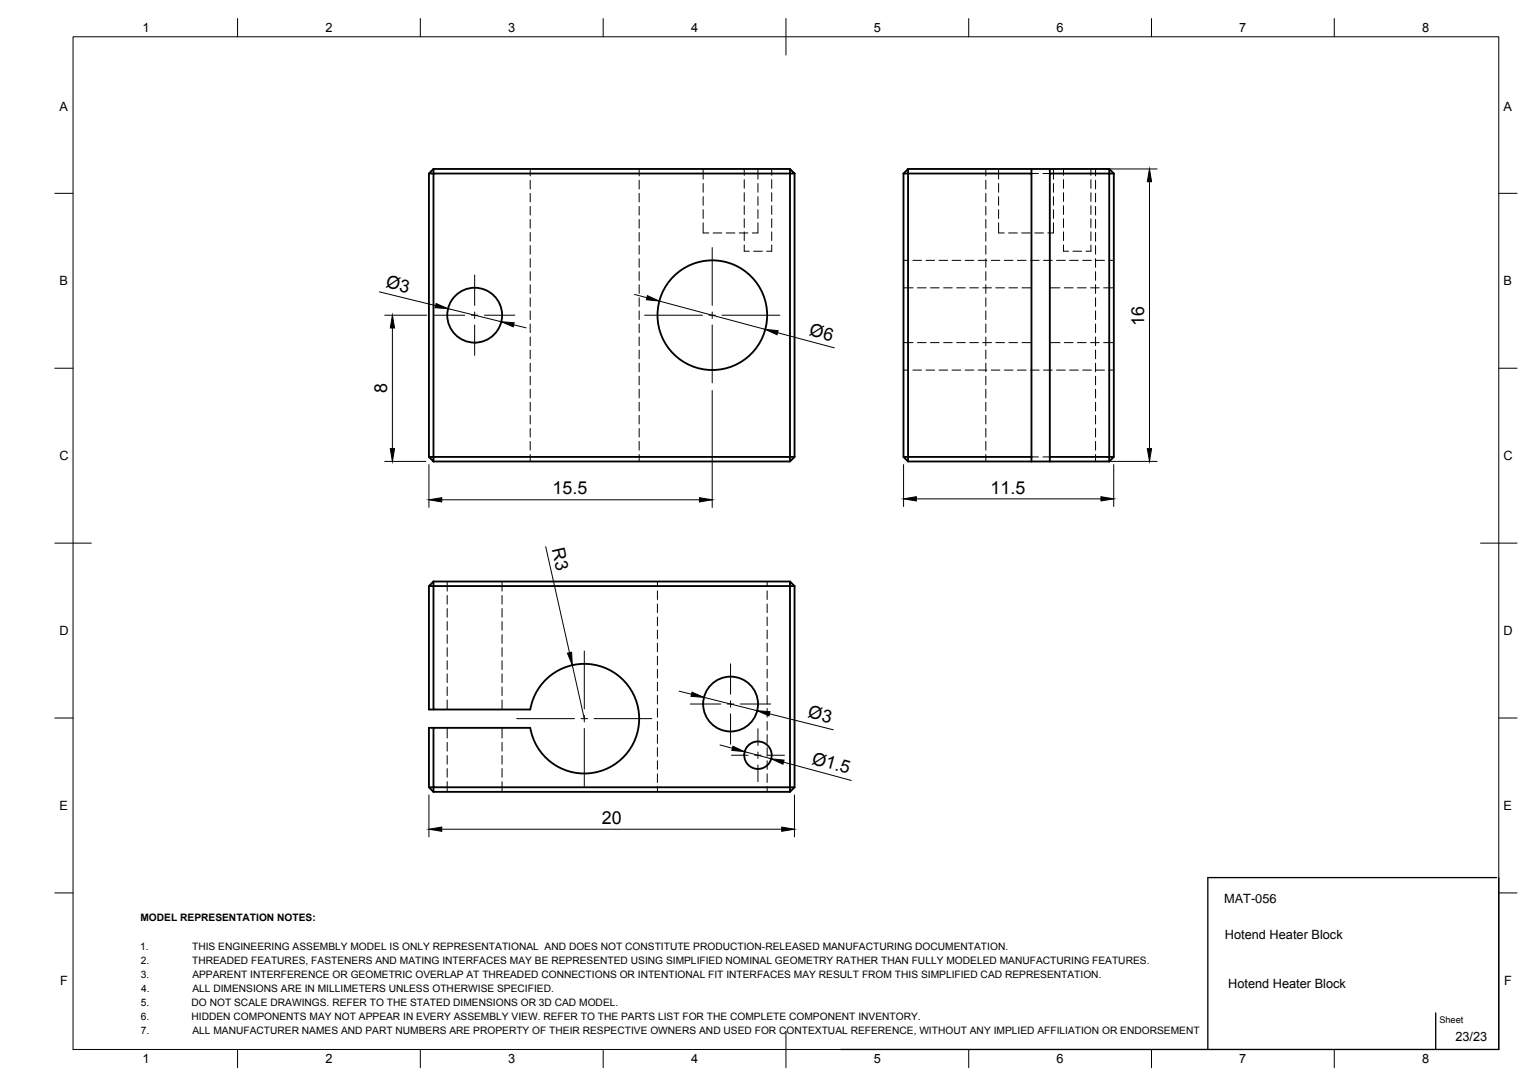
ISO-10303-21;
HEADER;
/* Generated by software containing ST-Developer
 * from STEP Tools, Inc. (www.steptools.com) 
 */

FILE_DESCRIPTION(
/* description */ (''),
/* implementation_level */ '2;1');

FILE_NAME(
/* name */ 'Hotend Heater Block.step',
/* time_stamp */ '2026-10-28T16:47:13+01:00',
/* author */ (''),
/* organization */ (''),
/* preprocessor_version */ 'ST-DEVELOPER v20.2',
/* originating_system */ 'Autodesk Translation Framework v15.17.0.0',
/* authorisation */ '');

FILE_SCHEMA (('AUTOMOTIVE_DESIGN { 1 0 10303 214 3 1 1 }'));
ENDSEC;

DATA;
#10=MECHANICAL_DESIGN_GEOMETRIC_PRESENTATION_REPRESENTATION('',(#4613),#459242);
#4425=SHAPE_REPRESENTATION_RELATIONSHIP('SRR','None',#459352,#4446);
#4446=ADVANCED_BREP_SHAPE_REPRESENTATION('',(#4493),#459241);
#4493=MANIFOLD_SOLID_BREP('E3D V6 heatblock',#94671);
#4613=STYLED_ITEM('',(#459505),#4493);
#5270=FACE_BOUND('',#18094,.T.);
#5271=FACE_BOUND('',#18095,.T.);
#5272=FACE_BOUND('',#18099,.T.);
#5273=FACE_BOUND('',#18100,.T.);
#5274=FACE_BOUND('',#18102,.T.);
#5275=FACE_BOUND('',#18103,.T.);
#5276=FACE_BOUND('',#18105,.T.);
#5277=FACE_BOUND('',#18107,.T.);
#6148=PLANE('',#105513);
#6149=PLANE('',#105514);
#6150=PLANE('',#105515);
#6151=PLANE('',#105516);
#6152=PLANE('',#105517);
#6153=PLANE('',#105518);
#6154=PLANE('',#105519);
#6155=PLANE('',#105520);
#6156=PLANE('',#105521);
#6157=PLANE('',#105522);
#6158=PLANE('',#105523);
#6159=PLANE('',#105524);
#6160=PLANE('',#105525);
#6161=PLANE('',#105526);
#6162=PLANE('',#105527);
#6163=PLANE('',#105528);
#6164=PLANE('',#105529);
#6165=PLANE('',#105530);
#6166=PLANE('',#105531);
#6167=PLANE('',#105532);
#6168=PLANE('',#105533);
#6169=PLANE('',#105534);
#6170=PLANE('',#105535);
#6171=PLANE('',#105536);
#6172=PLANE('',#105537);
#6173=PLANE('',#105538);
#6174=PLANE('',#105539);
#6175=PLANE('',#105540);
#6176=PLANE('',#105541);
#6177=PLANE('',#105542);
#6178=PLANE('',#105543);
#6179=PLANE('',#105544);
#6180=PLANE('',#105545);
#12120=FACE_OUTER_BOUND('',#18085,.T.);
#12121=FACE_OUTER_BOUND('',#18086,.T.);
#12122=FACE_OUTER_BOUND('',#18087,.T.);
#12123=FACE_OUTER_BOUND('',#18088,.T.);
#12124=FACE_OUTER_BOUND('',#18089,.T.);
#12125=FACE_OUTER_BOUND('',#18090,.T.);
#12126=FACE_OUTER_BOUND('',#18091,.T.);
#12127=FACE_OUTER_BOUND('',#18092,.T.);
#12128=FACE_OUTER_BOUND('',#18093,.T.);
#12129=FACE_OUTER_BOUND('',#18096,.T.);
#12130=FACE_OUTER_BOUND('',#18097,.T.);
#12131=FACE_OUTER_BOUND('',#18098,.T.);
#12132=FACE_OUTER_BOUND('',#18101,.T.);
#12133=FACE_OUTER_BOUND('',#18104,.T.);
#12134=FACE_OUTER_BOUND('',#18106,.T.);
#12135=FACE_OUTER_BOUND('',#18108,.T.);
#12136=FACE_OUTER_BOUND('',#18109,.T.);
#12137=FACE_OUTER_BOUND('',#18110,.T.);
#12138=FACE_OUTER_BOUND('',#18111,.T.);
#12139=FACE_OUTER_BOUND('',#18112,.T.);
#12140=FACE_OUTER_BOUND('',#18113,.T.);
#12141=FACE_OUTER_BOUND('',#18114,.T.);
#12142=FACE_OUTER_BOUND('',#18115,.T.);
#12143=FACE_OUTER_BOUND('',#18116,.T.);
#12144=FACE_OUTER_BOUND('',#18117,.T.);
#12145=FACE_OUTER_BOUND('',#18118,.T.);
#12146=FACE_OUTER_BOUND('',#18119,.T.);
#12147=FACE_OUTER_BOUND('',#18120,.T.);
#12148=FACE_OUTER_BOUND('',#18121,.T.);
#12149=FACE_OUTER_BOUND('',#18122,.T.);
#12150=FACE_OUTER_BOUND('',#18123,.T.);
#12151=FACE_OUTER_BOUND('',#18124,.T.);
#12152=FACE_OUTER_BOUND('',#18125,.T.);
#12153=FACE_OUTER_BOUND('',#18126,.T.);
#12154=FACE_OUTER_BOUND('',#18127,.T.);
#12155=FACE_OUTER_BOUND('',#18128,.T.);
#12156=FACE_OUTER_BOUND('',#18129,.T.);
#12157=FACE_OUTER_BOUND('',#18130,.T.);
#12158=FACE_OUTER_BOUND('',#18131,.T.);
#18085=EDGE_LOOP('',(#86890,#86891,#86892,#86893));
#18086=EDGE_LOOP('',(#86894,#86895,#86896,#86897));
#18087=EDGE_LOOP('',(#86898,#86899,#86900,#86901));
#18088=EDGE_LOOP('',(#86902,#86903,#86904,#86905));
#18089=EDGE_LOOP('',(#86906,#86907,#86908,#86909));
#18090=EDGE_LOOP('',(#86910,#86911,#86912,#86913));
#18091=EDGE_LOOP('',(#86914,#86915,#86916,#86917));
#18092=EDGE_LOOP('',(#86918,#86919,#86920,#86921));
#18093=EDGE_LOOP('',(#86922,#86923,#86924,#86925,#86926,#86927,#86928,#86929));
#18094=EDGE_LOOP('',(#86930));
#18095=EDGE_LOOP('',(#86931));
#18096=EDGE_LOOP('',(#86932,#86933,#86934,#86935));
#18097=EDGE_LOOP('',(#86936,#86937,#86938,#86939,#86940,#86941,#86942,#86943));
#18098=EDGE_LOOP('',(#86944,#86945,#86946,#86947));
#18099=EDGE_LOOP('',(#86948));
#18100=EDGE_LOOP('',(#86949));
#18101=EDGE_LOOP('',(#86950,#86951,#86952,#86953));
#18102=EDGE_LOOP('',(#86954));
#18103=EDGE_LOOP('',(#86955));
#18104=EDGE_LOOP('',(#86956,#86957,#86958,#86959,#86960,#86961));
#18105=EDGE_LOOP('',(#86962));
#18106=EDGE_LOOP('',(#86963,#86964,#86965,#86966,#86967,#86968));
#18107=EDGE_LOOP('',(#86969));
#18108=EDGE_LOOP('',(#86970));
#18109=EDGE_LOOP('',(#86971));
#18110=EDGE_LOOP('',(#86972,#86973,#86974,#86975));
#18111=EDGE_LOOP('',(#86976,#86977,#86978,#86979));
#18112=EDGE_LOOP('',(#86980,#86981,#86982));
#18113=EDGE_LOOP('',(#86983,#86984,#86985));
#18114=EDGE_LOOP('',(#86986,#86987,#86988,#86989));
#18115=EDGE_LOOP('',(#86990,#86991,#86992,#86993));
#18116=EDGE_LOOP('',(#86994,#86995,#86996,#86997));
#18117=EDGE_LOOP('',(#86998,#86999,#87000,#87001));
#18118=EDGE_LOOP('',(#87002,#87003,#87004,#87005));
#18119=EDGE_LOOP('',(#87006,#87007,#87008,#87009));
#18120=EDGE_LOOP('',(#87010,#87011,#87012,#87013));
#18121=EDGE_LOOP('',(#87014,#87015,#87016));
#18122=EDGE_LOOP('',(#87017,#87018,#87019));
#18123=EDGE_LOOP('',(#87020,#87021,#87022));
#18124=EDGE_LOOP('',(#87023,#87024,#87025));
#18125=EDGE_LOOP('',(#87026,#87027,#87028,#87029));
#18126=EDGE_LOOP('',(#87030,#87031,#87032,#87033));
#18127=EDGE_LOOP('',(#87034,#87035,#87036,#87037));
#18128=EDGE_LOOP('',(#87038,#87039,#87040,#87041));
#18129=EDGE_LOOP('',(#87042,#87043,#87044));
#18130=EDGE_LOOP('',(#87045,#87046,#87047));
#18131=EDGE_LOOP('',(#87048,#87049,#87050,#87051));
#23486=CIRCLE('',#105496,3.);
#23487=CIRCLE('',#105497,3.);
#23488=CIRCLE('',#105499,1.5);
#23489=CIRCLE('',#105500,1.5);
#23490=CIRCLE('',#105502,1.5);
#23491=CIRCLE('',#105503,1.5);
#23492=CIRCLE('',#105505,0.750000000000001);
#23493=CIRCLE('',#105506,0.750000000000001);
#23494=CIRCLE('',#105508,1.5);
#23495=CIRCLE('',#105509,1.5);
#23496=CIRCLE('',#105511,3.);
#23497=CIRCLE('',#105512,3.);
#30780=LINE('',#459000,#34582);
#30781=LINE('',#459006,#34583);
#30782=LINE('',#459012,#34584);
#30783=LINE('',#459018,#34585);
#30784=LINE('',#459024,#34586);
#30785=LINE('',#459031,#34587);
#30786=LINE('',#459034,#34588);
#30787=LINE('',#459038,#34589);
#30788=LINE('',#459040,#34590);
#30789=LINE('',#459042,#34591);
#30790=LINE('',#459043,#34592);
#30791=LINE('',#459047,#34593);
#30792=LINE('',#459049,#34594);
#30793=LINE('',#459051,#34595);
#30794=LINE('',#459052,#34596);
#30795=LINE('',#459055,#34597);
#30796=LINE('',#459057,#34598);
#30797=LINE('',#459059,#34599);
#30798=LINE('',#459061,#34600);
#30799=LINE('',#459063,#34601);
#30800=LINE('',#459065,#34602);
#30801=LINE('',#459066,#34603);
#30802=LINE('',#459070,#34604);
#30803=LINE('',#459072,#34605);
#30804=LINE('',#459074,#34606);
#30805=LINE('',#459075,#34607);
#30806=LINE('',#459079,#34608);
#30807=LINE('',#459081,#34609);
#30808=LINE('',#459082,#34610);
#30809=LINE('',#459084,#34611);
#30810=LINE('',#459086,#34612);
#30811=LINE('',#459088,#34613);
#30812=LINE('',#459089,#34614);
#30813=LINE('',#459093,#34615);
#30814=LINE('',#459095,#34616);
#30815=LINE('',#459097,#34617);
#30816=LINE('',#459098,#34618);
#30817=LINE('',#459102,#34619);
#30818=LINE('',#459104,#34620);
#30819=LINE('',#459106,#34621);
#30820=LINE('',#459107,#34622);
#30821=LINE('',#459109,#34623);
#30822=LINE('',#459110,#34624);
#30823=LINE('',#459112,#34625);
#30824=LINE('',#459113,#34626);
#30825=LINE('',#459117,#34627);
#30826=LINE('',#459119,#34628);
#30827=LINE('',#459121,#34629);
#30828=LINE('',#459122,#34630);
#30829=LINE('',#459124,#34631);
#30830=LINE('',#459125,#34632);
#30831=LINE('',#459127,#34633);
#30832=LINE('',#459129,#34634);
#30833=LINE('',#459131,#34635);
#30834=LINE('',#459133,#34636);
#30835=LINE('',#459134,#34637);
#30836=LINE('',#459136,#34638);
#30837=LINE('',#459138,#34639);
#30838=LINE('',#459140,#34640);
#30839=LINE('',#459142,#34641);
#30840=LINE('',#459144,#34642);
#30841=LINE('',#459146,#34643);
#30842=LINE('',#459148,#34644);
#30843=LINE('',#459150,#34645);
#30844=LINE('',#459152,#34646);
#30845=LINE('',#459154,#34647);
#30846=LINE('',#459156,#34648);
#30847=LINE('',#459158,#34649);
#30848=LINE('',#459160,#34650);
#34582=VECTOR('',#130494,3.);
#34583=VECTOR('',#130501,1.5);
#34584=VECTOR('',#130508,1.5);
#34585=VECTOR('',#130515,0.750000000000001);
#34586=VECTOR('',#130522,1.5);
#34587=VECTOR('',#130529,1000.);
#34588=VECTOR('',#130532,1000.);
#34589=VECTOR('',#130535,1000.);
#34590=VECTOR('',#130536,1000.);
#34591=VECTOR('',#130537,1000.);
#34592=VECTOR('',#130538,1000.);
#34593=VECTOR('',#130541,1000.);
#34594=VECTOR('',#130542,1000.);
#34595=VECTOR('',#130543,1000.);
#34596=VECTOR('',#130544,1000.);
#34597=VECTOR('',#130547,1000.);
#34598=VECTOR('',#130548,1000.);
#34599=VECTOR('',#130549,1000.);
#34600=VECTOR('',#130550,1000.);
#34601=VECTOR('',#130551,1000.);
#34602=VECTOR('',#130552,1000.);
#34603=VECTOR('',#130553,1000.);
#34604=VECTOR('',#130556,1000.);
#34605=VECTOR('',#130557,1000.);
#34606=VECTOR('',#130558,1000.);
#34607=VECTOR('',#130559,1000.);
#34608=VECTOR('',#130562,1000.);
#34609=VECTOR('',#130563,1000.);
#34610=VECTOR('',#130564,1000.);
#34611=VECTOR('',#130565,1000.);
#34612=VECTOR('',#130566,1000.);
#34613=VECTOR('',#130567,1000.);
#34614=VECTOR('',#130568,1000.);
#34615=VECTOR('',#130571,1000.);
#34616=VECTOR('',#130572,1000.);
#34617=VECTOR('',#130573,1000.);
#34618=VECTOR('',#130574,1000.);
#34619=VECTOR('',#130577,1000.);
#34620=VECTOR('',#130578,1000.);
#34621=VECTOR('',#130579,1000.);
#34622=VECTOR('',#130580,1000.);
#34623=VECTOR('',#130583,1000.);
#34624=VECTOR('',#130584,1000.);
#34625=VECTOR('',#130587,1000.);
#34626=VECTOR('',#130588,1000.);
#34627=VECTOR('',#130595,1000.);
#34628=VECTOR('',#130598,1000.);
#34629=VECTOR('',#130601,1000.);
#34630=VECTOR('',#130602,1000.);
#34631=VECTOR('',#130605,1000.);
#34632=VECTOR('',#130606,1000.);
#34633=VECTOR('',#130609,1000.);
#34634=VECTOR('',#130612,1000.);
#34635=VECTOR('',#130615,1000.);
#34636=VECTOR('',#130618,1000.);
#34637=VECTOR('',#130619,1000.);
#34638=VECTOR('',#130622,1000.);
#34639=VECTOR('',#130625,1000.);
#34640=VECTOR('',#130628,1000.);
#34641=VECTOR('',#130631,1000.);
#34642=VECTOR('',#130634,1000.);
#34643=VECTOR('',#130637,1000.);
#34644=VECTOR('',#130640,1000.);
#34645=VECTOR('',#130643,1000.);
#34646=VECTOR('',#130646,1000.);
#34647=VECTOR('',#130649,1000.);
#34648=VECTOR('',#130652,1000.);
#34649=VECTOR('',#130655,1000.);
#34650=VECTOR('',#130658,1000.);
#43470=VERTEX_POINT('',#458997);
#43471=VERTEX_POINT('',#458999);
#43472=VERTEX_POINT('',#459003);
#43473=VERTEX_POINT('',#459005);
#43474=VERTEX_POINT('',#459009);
#43475=VERTEX_POINT('',#459011);
#43476=VERTEX_POINT('',#459015);
#43477=VERTEX_POINT('',#459017);
#43478=VERTEX_POINT('',#459021);
#43479=VERTEX_POINT('',#459023);
#43480=VERTEX_POINT('',#459027);
#43481=VERTEX_POINT('',#459028);
#43482=VERTEX_POINT('',#459030);
#43483=VERTEX_POINT('',#459032);
#43484=VERTEX_POINT('',#459036);
#43485=VERTEX_POINT('',#459037);
#43486=VERTEX_POINT('',#459039);
#43487=VERTEX_POINT('',#459041);
#43488=VERTEX_POINT('',#459045);
#43489=VERTEX_POINT('',#459046);
#43490=VERTEX_POINT('',#459048);
#43491=VERTEX_POINT('',#459050);
#43492=VERTEX_POINT('',#459054);
#43493=VERTEX_POINT('',#459056);
#43494=VERTEX_POINT('',#459058);
#43495=VERTEX_POINT('',#459060);
#43496=VERTEX_POINT('',#459062);
#43497=VERTEX_POINT('',#459064);
#43498=VERTEX_POINT('',#459068);
#43499=VERTEX_POINT('',#459069);
#43500=VERTEX_POINT('',#459071);
#43501=VERTEX_POINT('',#459073);
#43502=VERTEX_POINT('',#459077);
#43503=VERTEX_POINT('',#459078);
#43504=VERTEX_POINT('',#459080);
#43505=VERTEX_POINT('',#459083);
#43506=VERTEX_POINT('',#459085);
#43507=VERTEX_POINT('',#459087);
#43508=VERTEX_POINT('',#459091);
#43509=VERTEX_POINT('',#459092);
#43510=VERTEX_POINT('',#459094);
#43511=VERTEX_POINT('',#459096);
#43512=VERTEX_POINT('',#459100);
#43513=VERTEX_POINT('',#459101);
#43514=VERTEX_POINT('',#459103);
#43515=VERTEX_POINT('',#459105);
#57947=EDGE_CURVE('',#43470,#43470,#23486,.T.);
#57948=EDGE_CURVE('',#43470,#43471,#30780,.T.);
#57949=EDGE_CURVE('',#43471,#43471,#23487,.T.);
#57950=EDGE_CURVE('',#43472,#43472,#23488,.T.);
#57951=EDGE_CURVE('',#43472,#43473,#30781,.T.);
#57952=EDGE_CURVE('',#43473,#43473,#23489,.T.);
#57953=EDGE_CURVE('',#43474,#43474,#23490,.T.);
#57954=EDGE_CURVE('',#43474,#43475,#30782,.T.);
#57955=EDGE_CURVE('',#43475,#43475,#23491,.T.);
#57956=EDGE_CURVE('',#43476,#43476,#23492,.T.);
#57957=EDGE_CURVE('',#43476,#43477,#30783,.T.);
#57958=EDGE_CURVE('',#43477,#43477,#23493,.T.);
#57959=EDGE_CURVE('',#43478,#43478,#23494,.T.);
#57960=EDGE_CURVE('',#43478,#43479,#30784,.T.);
#57961=EDGE_CURVE('',#43479,#43479,#23495,.T.);
#57962=EDGE_CURVE('',#43480,#43481,#23496,.T.);
#57963=EDGE_CURVE('',#43480,#43482,#30785,.T.);
#57964=EDGE_CURVE('',#43482,#43483,#23497,.T.);
#57965=EDGE_CURVE('',#43481,#43483,#30786,.T.);
#57966=EDGE_CURVE('',#43484,#43485,#30787,.T.);
#57967=EDGE_CURVE('',#43485,#43486,#30788,.T.);
#57968=EDGE_CURVE('',#43487,#43486,#30789,.T.);
#57969=EDGE_CURVE('',#43487,#43484,#30790,.T.);
#57970=EDGE_CURVE('',#43488,#43489,#30791,.T.);
#57971=EDGE_CURVE('',#43489,#43490,#30792,.T.);
#57972=EDGE_CURVE('',#43490,#43491,#30793,.T.);
#57973=EDGE_CURVE('',#43491,#43488,#30794,.T.);
#57974=EDGE_CURVE('',#43492,#43482,#30795,.T.);
#57975=EDGE_CURVE('',#43492,#43493,#30796,.T.);
#57976=EDGE_CURVE('',#43493,#43494,#30797,.T.);
#57977=EDGE_CURVE('',#43494,#43495,#30798,.T.);
#57978=EDGE_CURVE('',#43495,#43496,#30799,.T.);
#57979=EDGE_CURVE('',#43496,#43497,#30800,.T.);
#57980=EDGE_CURVE('',#43483,#43497,#30801,.T.);
#57981=EDGE_CURVE('',#43498,#43499,#30802,.T.);
#57982=EDGE_CURVE('',#43499,#43500,#30803,.T.);
#57983=EDGE_CURVE('',#43500,#43501,#30804,.T.);
#57984=EDGE_CURVE('',#43501,#43498,#30805,.T.);
#57985=EDGE_CURVE('',#43502,#43503,#30806,.T.);
#57986=EDGE_CURVE('',#43503,#43504,#30807,.T.);
#57987=EDGE_CURVE('',#43504,#43480,#30808,.T.);
#57988=EDGE_CURVE('',#43481,#43505,#30809,.T.);
#57989=EDGE_CURVE('',#43505,#43506,#30810,.T.);
#57990=EDGE_CURVE('',#43506,#43507,#30811,.T.);
#57991=EDGE_CURVE('',#43507,#43502,#30812,.T.);
#57992=EDGE_CURVE('',#43508,#43509,#30813,.T.);
#57993=EDGE_CURVE('',#43509,#43510,#30814,.T.);
#57994=EDGE_CURVE('',#43510,#43511,#30815,.T.);
#57995=EDGE_CURVE('',#43511,#43508,#30816,.T.);
#57996=EDGE_CURVE('',#43512,#43513,#30817,.T.);
#57997=EDGE_CURVE('',#43513,#43514,#30818,.T.);
#57998=EDGE_CURVE('',#43514,#43515,#30819,.T.);
#57999=EDGE_CURVE('',#43515,#43512,#30820,.T.);
#58000=EDGE_CURVE('',#43486,#43492,#30821,.T.);
#58001=EDGE_CURVE('',#43504,#43487,#30822,.T.);
#58002=EDGE_CURVE('',#43497,#43489,#30823,.T.);
#58003=EDGE_CURVE('',#43488,#43505,#30824,.T.);
#58004=EDGE_CURVE('',#43506,#43491,#30825,.T.);
#58005=EDGE_CURVE('',#43484,#43503,#30826,.T.);
#58006=EDGE_CURVE('',#43506,#43511,#30827,.T.);
#58007=EDGE_CURVE('',#43511,#43491,#30828,.T.);
#58008=EDGE_CURVE('',#43484,#43512,#30829,.T.);
#58009=EDGE_CURVE('',#43512,#43503,#30830,.T.);
#58010=EDGE_CURVE('',#43490,#43496,#30831,.T.);
#58011=EDGE_CURVE('',#43508,#43490,#30832,.T.);
#58012=EDGE_CURVE('',#43507,#43510,#30833,.T.);
#58013=EDGE_CURVE('',#43502,#43501,#30834,.T.);
#58014=EDGE_CURVE('',#43498,#43507,#30835,.T.);
#58015=EDGE_CURVE('',#43513,#43502,#30836,.T.);
#58016=EDGE_CURVE('',#43485,#43515,#30837,.T.);
#58017=EDGE_CURVE('',#43493,#43485,#30838,.T.);
#58018=EDGE_CURVE('',#43508,#43496,#30839,.T.);
#58019=EDGE_CURVE('',#43498,#43510,#30840,.T.);
#58020=EDGE_CURVE('',#43513,#43501,#30841,.T.);
#58021=EDGE_CURVE('',#43493,#43515,#30842,.T.);
#58022=EDGE_CURVE('',#43509,#43495,#30843,.T.);
#58023=EDGE_CURVE('',#43499,#43509,#30844,.T.);
#58024=EDGE_CURVE('',#43514,#43500,#30845,.T.);
#58025=EDGE_CURVE('',#43494,#43514,#30846,.T.);
#58026=EDGE_CURVE('',#43499,#43495,#30847,.T.);
#58027=EDGE_CURVE('',#43494,#43500,#30848,.T.);
#86890=ORIENTED_EDGE('',*,*,#57947,.F.);
#86891=ORIENTED_EDGE('',*,*,#57948,.T.);
#86892=ORIENTED_EDGE('',*,*,#57949,.T.);
#86893=ORIENTED_EDGE('',*,*,#57948,.F.);
#86894=ORIENTED_EDGE('',*,*,#57950,.F.);
#86895=ORIENTED_EDGE('',*,*,#57951,.T.);
#86896=ORIENTED_EDGE('',*,*,#57952,.F.);
#86897=ORIENTED_EDGE('',*,*,#57951,.F.);
#86898=ORIENTED_EDGE('',*,*,#57953,.F.);
#86899=ORIENTED_EDGE('',*,*,#57954,.T.);
#86900=ORIENTED_EDGE('',*,*,#57955,.T.);
#86901=ORIENTED_EDGE('',*,*,#57954,.F.);
#86902=ORIENTED_EDGE('',*,*,#57956,.F.);
#86903=ORIENTED_EDGE('',*,*,#57957,.T.);
#86904=ORIENTED_EDGE('',*,*,#57958,.T.);
#86905=ORIENTED_EDGE('',*,*,#57957,.F.);
#86906=ORIENTED_EDGE('',*,*,#57959,.F.);
#86907=ORIENTED_EDGE('',*,*,#57960,.T.);
#86908=ORIENTED_EDGE('',*,*,#57961,.T.);
#86909=ORIENTED_EDGE('',*,*,#57960,.F.);
#86910=ORIENTED_EDGE('',*,*,#57962,.F.);
#86911=ORIENTED_EDGE('',*,*,#57963,.T.);
#86912=ORIENTED_EDGE('',*,*,#57964,.T.);
#86913=ORIENTED_EDGE('',*,*,#57965,.F.);
#86914=ORIENTED_EDGE('',*,*,#57966,.T.);
#86915=ORIENTED_EDGE('',*,*,#57967,.T.);
#86916=ORIENTED_EDGE('',*,*,#57968,.F.);
#86917=ORIENTED_EDGE('',*,*,#57969,.T.);
#86918=ORIENTED_EDGE('',*,*,#57970,.T.);
#86919=ORIENTED_EDGE('',*,*,#57971,.T.);
#86920=ORIENTED_EDGE('',*,*,#57972,.T.);
#86921=ORIENTED_EDGE('',*,*,#57973,.T.);
#86922=ORIENTED_EDGE('',*,*,#57974,.F.);
#86923=ORIENTED_EDGE('',*,*,#57975,.T.);
#86924=ORIENTED_EDGE('',*,*,#57976,.T.);
#86925=ORIENTED_EDGE('',*,*,#57977,.T.);
#86926=ORIENTED_EDGE('',*,*,#57978,.T.);
#86927=ORIENTED_EDGE('',*,*,#57979,.T.);
#86928=ORIENTED_EDGE('',*,*,#57980,.F.);
#86929=ORIENTED_EDGE('',*,*,#57964,.F.);
#86930=ORIENTED_EDGE('',*,*,#57958,.F.);
#86931=ORIENTED_EDGE('',*,*,#57961,.F.);
#86932=ORIENTED_EDGE('',*,*,#57981,.T.);
#86933=ORIENTED_EDGE('',*,*,#57982,.T.);
#86934=ORIENTED_EDGE('',*,*,#57983,.T.);
#86935=ORIENTED_EDGE('',*,*,#57984,.T.);
#86936=ORIENTED_EDGE('',*,*,#57985,.T.);
#86937=ORIENTED_EDGE('',*,*,#57986,.T.);
#86938=ORIENTED_EDGE('',*,*,#57987,.T.);
#86939=ORIENTED_EDGE('',*,*,#57962,.T.);
#86940=ORIENTED_EDGE('',*,*,#57988,.T.);
#86941=ORIENTED_EDGE('',*,*,#57989,.T.);
#86942=ORIENTED_EDGE('',*,*,#57990,.T.);
#86943=ORIENTED_EDGE('',*,*,#57991,.T.);
#86944=ORIENTED_EDGE('',*,*,#57992,.T.);
#86945=ORIENTED_EDGE('',*,*,#57993,.T.);
#86946=ORIENTED_EDGE('',*,*,#57994,.T.);
#86947=ORIENTED_EDGE('',*,*,#57995,.T.);
#86948=ORIENTED_EDGE('',*,*,#57949,.F.);
#86949=ORIENTED_EDGE('',*,*,#57955,.F.);
#86950=ORIENTED_EDGE('',*,*,#57996,.T.);
#86951=ORIENTED_EDGE('',*,*,#57997,.T.);
#86952=ORIENTED_EDGE('',*,*,#57998,.T.);
#86953=ORIENTED_EDGE('',*,*,#57999,.T.);
#86954=ORIENTED_EDGE('',*,*,#57947,.T.);
#86955=ORIENTED_EDGE('',*,*,#57950,.T.);
#86956=ORIENTED_EDGE('',*,*,#57968,.T.);
#86957=ORIENTED_EDGE('',*,*,#58000,.T.);
#86958=ORIENTED_EDGE('',*,*,#57974,.T.);
#86959=ORIENTED_EDGE('',*,*,#57963,.F.);
#86960=ORIENTED_EDGE('',*,*,#57987,.F.);
#86961=ORIENTED_EDGE('',*,*,#58001,.T.);
#86962=ORIENTED_EDGE('',*,*,#57952,.T.);
#86963=ORIENTED_EDGE('',*,*,#57980,.T.);
#86964=ORIENTED_EDGE('',*,*,#58002,.T.);
#86965=ORIENTED_EDGE('',*,*,#57970,.F.);
#86966=ORIENTED_EDGE('',*,*,#58003,.T.);
#86967=ORIENTED_EDGE('',*,*,#57988,.F.);
#86968=ORIENTED_EDGE('',*,*,#57965,.T.);
#86969=ORIENTED_EDGE('',*,*,#57953,.T.);
#86970=ORIENTED_EDGE('',*,*,#57959,.T.);
#86971=ORIENTED_EDGE('',*,*,#57956,.T.);
#86972=ORIENTED_EDGE('',*,*,#58003,.F.);
#86973=ORIENTED_EDGE('',*,*,#57973,.F.);
#86974=ORIENTED_EDGE('',*,*,#58004,.F.);
#86975=ORIENTED_EDGE('',*,*,#57989,.F.);
#86976=ORIENTED_EDGE('',*,*,#58001,.F.);
#86977=ORIENTED_EDGE('',*,*,#57986,.F.);
#86978=ORIENTED_EDGE('',*,*,#58005,.F.);
#86979=ORIENTED_EDGE('',*,*,#57969,.F.);
#86980=ORIENTED_EDGE('',*,*,#58006,.F.);
#86981=ORIENTED_EDGE('',*,*,#58004,.T.);
#86982=ORIENTED_EDGE('',*,*,#58007,.F.);
#86983=ORIENTED_EDGE('',*,*,#58008,.F.);
#86984=ORIENTED_EDGE('',*,*,#58005,.T.);
#86985=ORIENTED_EDGE('',*,*,#58009,.F.);
#86986=ORIENTED_EDGE('',*,*,#58002,.F.);
#86987=ORIENTED_EDGE('',*,*,#57979,.F.);
#86988=ORIENTED_EDGE('',*,*,#58010,.F.);
#86989=ORIENTED_EDGE('',*,*,#57971,.F.);
#86990=ORIENTED_EDGE('',*,*,#58007,.T.);
#86991=ORIENTED_EDGE('',*,*,#57972,.F.);
#86992=ORIENTED_EDGE('',*,*,#58011,.F.);
#86993=ORIENTED_EDGE('',*,*,#57995,.F.);
#86994=ORIENTED_EDGE('',*,*,#58006,.T.);
#86995=ORIENTED_EDGE('',*,*,#57994,.F.);
#86996=ORIENTED_EDGE('',*,*,#58012,.F.);
#86997=ORIENTED_EDGE('',*,*,#57990,.F.);
#86998=ORIENTED_EDGE('',*,*,#58013,.F.);
#86999=ORIENTED_EDGE('',*,*,#57991,.F.);
#87000=ORIENTED_EDGE('',*,*,#58014,.F.);
#87001=ORIENTED_EDGE('',*,*,#57984,.F.);
#87002=ORIENTED_EDGE('',*,*,#58009,.T.);
#87003=ORIENTED_EDGE('',*,*,#57985,.F.);
#87004=ORIENTED_EDGE('',*,*,#58015,.F.);
#87005=ORIENTED_EDGE('',*,*,#57996,.F.);
#87006=ORIENTED_EDGE('',*,*,#58008,.T.);
#87007=ORIENTED_EDGE('',*,*,#57999,.F.);
#87008=ORIENTED_EDGE('',*,*,#58016,.F.);
#87009=ORIENTED_EDGE('',*,*,#57966,.F.);
#87010=ORIENTED_EDGE('',*,*,#58000,.F.);
#87011=ORIENTED_EDGE('',*,*,#57967,.F.);
#87012=ORIENTED_EDGE('',*,*,#58017,.F.);
#87013=ORIENTED_EDGE('',*,*,#57975,.F.);
#87014=ORIENTED_EDGE('',*,*,#58011,.T.);
#87015=ORIENTED_EDGE('',*,*,#58010,.T.);
#87016=ORIENTED_EDGE('',*,*,#58018,.F.);
#87017=ORIENTED_EDGE('',*,*,#58014,.T.);
#87018=ORIENTED_EDGE('',*,*,#58012,.T.);
#87019=ORIENTED_EDGE('',*,*,#58019,.F.);
#87020=ORIENTED_EDGE('',*,*,#58015,.T.);
#87021=ORIENTED_EDGE('',*,*,#58013,.T.);
#87022=ORIENTED_EDGE('',*,*,#58020,.F.);
#87023=ORIENTED_EDGE('',*,*,#58017,.T.);
#87024=ORIENTED_EDGE('',*,*,#58016,.T.);
#87025=ORIENTED_EDGE('',*,*,#58021,.F.);
#87026=ORIENTED_EDGE('',*,*,#58018,.T.);
#87027=ORIENTED_EDGE('',*,*,#57978,.F.);
#87028=ORIENTED_EDGE('',*,*,#58022,.F.);
#87029=ORIENTED_EDGE('',*,*,#57992,.F.);
#87030=ORIENTED_EDGE('',*,*,#58019,.T.);
#87031=ORIENTED_EDGE('',*,*,#57993,.F.);
#87032=ORIENTED_EDGE('',*,*,#58023,.F.);
#87033=ORIENTED_EDGE('',*,*,#57981,.F.);
#87034=ORIENTED_EDGE('',*,*,#58020,.T.);
#87035=ORIENTED_EDGE('',*,*,#57983,.F.);
#87036=ORIENTED_EDGE('',*,*,#58024,.F.);
#87037=ORIENTED_EDGE('',*,*,#57997,.F.);
#87038=ORIENTED_EDGE('',*,*,#58021,.T.);
#87039=ORIENTED_EDGE('',*,*,#57998,.F.);
#87040=ORIENTED_EDGE('',*,*,#58025,.F.);
#87041=ORIENTED_EDGE('',*,*,#57976,.F.);
#87042=ORIENTED_EDGE('',*,*,#58023,.T.);
#87043=ORIENTED_EDGE('',*,*,#58022,.T.);
#87044=ORIENTED_EDGE('',*,*,#58026,.F.);
#87045=ORIENTED_EDGE('',*,*,#58025,.T.);
#87046=ORIENTED_EDGE('',*,*,#58024,.T.);
#87047=ORIENTED_EDGE('',*,*,#58027,.F.);
#87048=ORIENTED_EDGE('',*,*,#58026,.T.);
#87049=ORIENTED_EDGE('',*,*,#57977,.F.);
#87050=ORIENTED_EDGE('',*,*,#58027,.T.);
#87051=ORIENTED_EDGE('',*,*,#57982,.F.);
#88809=CYLINDRICAL_SURFACE('',#105495,3.);
#88810=CYLINDRICAL_SURFACE('',#105498,1.5);
#88811=CYLINDRICAL_SURFACE('',#105501,1.5);
#88812=CYLINDRICAL_SURFACE('',#105504,0.750000000000001);
#88813=CYLINDRICAL_SURFACE('',#105507,1.5);
#88814=CYLINDRICAL_SURFACE('',#105510,3.);
#94584=ADVANCED_FACE('',(#12120),#88809,.F.);
#94585=ADVANCED_FACE('',(#12121),#88810,.F.);
#94586=ADVANCED_FACE('',(#12122),#88811,.F.);
#94587=ADVANCED_FACE('',(#12123),#88812,.F.);
#94588=ADVANCED_FACE('',(#12124),#88813,.F.);
#94589=ADVANCED_FACE('',(#12125),#88814,.F.);
#94590=ADVANCED_FACE('',(#12126),#6148,.F.);
#94591=ADVANCED_FACE('',(#12127),#6149,.F.);
#94592=ADVANCED_FACE('',(#12128,#5270,#5271),#6150,.F.);
#94593=ADVANCED_FACE('',(#12129),#6151,.F.);
#94594=ADVANCED_FACE('',(#12130),#6152,.F.);
#94595=ADVANCED_FACE('',(#12131,#5272,#5273),#6153,.T.);
#94596=ADVANCED_FACE('',(#12132,#5274,#5275),#6154,.F.);
#94597=ADVANCED_FACE('',(#12133,#5276),#6155,.F.);
#94598=ADVANCED_FACE('',(#12134,#5277),#6156,.F.);
#94599=ADVANCED_FACE('',(#12135),#6157,.T.);
#94600=ADVANCED_FACE('',(#12136),#6158,.T.);
#94601=ADVANCED_FACE('',(#12137),#6159,.F.);
#94602=ADVANCED_FACE('',(#12138),#6160,.F.);
#94603=ADVANCED_FACE('',(#12139),#6161,.T.);
#94604=ADVANCED_FACE('',(#12140),#6162,.T.);
#94605=ADVANCED_FACE('',(#12141),#6163,.F.);
#94606=ADVANCED_FACE('',(#12142),#6164,.T.);
#94607=ADVANCED_FACE('',(#12143),#6165,.T.);
#94608=ADVANCED_FACE('',(#12144),#6166,.F.);
#94609=ADVANCED_FACE('',(#12145),#6167,.F.);
#94610=ADVANCED_FACE('',(#12146),#6168,.F.);
#94611=ADVANCED_FACE('',(#12147),#6169,.F.);
#94612=ADVANCED_FACE('',(#12148),#6170,.T.);
#94613=ADVANCED_FACE('',(#12149),#6171,.T.);
#94614=ADVANCED_FACE('',(#12150),#6172,.T.);
#94615=ADVANCED_FACE('',(#12151),#6173,.T.);
#94616=ADVANCED_FACE('',(#12152),#6174,.T.);
#94617=ADVANCED_FACE('',(#12153),#6175,.T.);
#94618=ADVANCED_FACE('',(#12154),#6176,.F.);
#94619=ADVANCED_FACE('',(#12155),#6177,.F.);
#94620=ADVANCED_FACE('',(#12156),#6178,.T.);
#94621=ADVANCED_FACE('',(#12157),#6179,.T.);
#94622=ADVANCED_FACE('',(#12158),#6180,.F.);
#94671=CLOSED_SHELL('',(#94584,#94585,#94586,#94587,#94588,#94589,#94590,
#94591,#94592,#94593,#94594,#94595,#94596,#94597,#94598,#94599,#94600,#94601,
#94602,#94603,#94604,#94605,#94606,#94607,#94608,#94609,#94610,#94611,#94612,
#94613,#94614,#94615,#94616,#94617,#94618,#94619,#94620,#94621,#94622));
#105494=AXIS2_PLACEMENT_3D('',#458995,#130488,#130489);
#105495=AXIS2_PLACEMENT_3D('',#458996,#130490,#130491);
#105496=AXIS2_PLACEMENT_3D('',#458998,#130492,#130493);
#105497=AXIS2_PLACEMENT_3D('',#459001,#130495,#130496);
#105498=AXIS2_PLACEMENT_3D('',#459002,#130497,#130498);
#105499=AXIS2_PLACEMENT_3D('',#459004,#130499,#130500);
#105500=AXIS2_PLACEMENT_3D('',#459007,#130502,#130503);
#105501=AXIS2_PLACEMENT_3D('',#459008,#130504,#130505);
#105502=AXIS2_PLACEMENT_3D('',#459010,#130506,#130507);
#105503=AXIS2_PLACEMENT_3D('',#459013,#130509,#130510);
#105504=AXIS2_PLACEMENT_3D('',#459014,#130511,#130512);
#105505=AXIS2_PLACEMENT_3D('',#459016,#130513,#130514);
#105506=AXIS2_PLACEMENT_3D('',#459019,#130516,#130517);
#105507=AXIS2_PLACEMENT_3D('',#459020,#130518,#130519);
#105508=AXIS2_PLACEMENT_3D('',#459022,#130520,#130521);
#105509=AXIS2_PLACEMENT_3D('',#459025,#130523,#130524);
#105510=AXIS2_PLACEMENT_3D('',#459026,#130525,#130526);
#105511=AXIS2_PLACEMENT_3D('',#459029,#130527,#130528);
#105512=AXIS2_PLACEMENT_3D('',#459033,#130530,#130531);
#105513=AXIS2_PLACEMENT_3D('',#459035,#130533,#130534);
#105514=AXIS2_PLACEMENT_3D('',#459044,#130539,#130540);
#105515=AXIS2_PLACEMENT_3D('',#459053,#130545,#130546);
#105516=AXIS2_PLACEMENT_3D('',#459067,#130554,#130555);
#105517=AXIS2_PLACEMENT_3D('',#459076,#130560,#130561);
#105518=AXIS2_PLACEMENT_3D('',#459090,#130569,#130570);
#105519=AXIS2_PLACEMENT_3D('',#459099,#130575,#130576);
#105520=AXIS2_PLACEMENT_3D('',#459108,#130581,#130582);
#105521=AXIS2_PLACEMENT_3D('',#459111,#130585,#130586);
#105522=AXIS2_PLACEMENT_3D('',#459114,#130589,#130590);
#105523=AXIS2_PLACEMENT_3D('',#459115,#130591,#130592);
#105524=AXIS2_PLACEMENT_3D('',#459116,#130593,#130594);
#105525=AXIS2_PLACEMENT_3D('',#459118,#130596,#130597);
#105526=AXIS2_PLACEMENT_3D('',#459120,#130599,#130600);
#105527=AXIS2_PLACEMENT_3D('',#459123,#130603,#130604);
#105528=AXIS2_PLACEMENT_3D('',#459126,#130607,#130608);
#105529=AXIS2_PLACEMENT_3D('',#459128,#130610,#130611);
#105530=AXIS2_PLACEMENT_3D('',#459130,#130613,#130614);
#105531=AXIS2_PLACEMENT_3D('',#459132,#130616,#130617);
#105532=AXIS2_PLACEMENT_3D('',#459135,#130620,#130621);
#105533=AXIS2_PLACEMENT_3D('',#459137,#130623,#130624);
#105534=AXIS2_PLACEMENT_3D('',#459139,#130626,#130627);
#105535=AXIS2_PLACEMENT_3D('',#459141,#130629,#130630);
#105536=AXIS2_PLACEMENT_3D('',#459143,#130632,#130633);
#105537=AXIS2_PLACEMENT_3D('',#459145,#130635,#130636);
#105538=AXIS2_PLACEMENT_3D('',#459147,#130638,#130639);
#105539=AXIS2_PLACEMENT_3D('',#459149,#130641,#130642);
#105540=AXIS2_PLACEMENT_3D('',#459151,#130644,#130645);
#105541=AXIS2_PLACEMENT_3D('',#459153,#130647,#130648);
#105542=AXIS2_PLACEMENT_3D('',#459155,#130650,#130651);
#105543=AXIS2_PLACEMENT_3D('',#459157,#130653,#130654);
#105544=AXIS2_PLACEMENT_3D('',#459159,#130656,#130657);
#105545=AXIS2_PLACEMENT_3D('',#459161,#130659,#130660);
#130488=DIRECTION('axis',(0.,0.,1.));
#130489=DIRECTION('refdir',(1.,0.,0.));
#130490=DIRECTION('center_axis',(0.,1.,0.));
#130491=DIRECTION('ref_axis',(0.,0.,1.));
#130492=DIRECTION('center_axis',(0.,1.,0.));
#130493=DIRECTION('ref_axis',(0.,0.,1.));
#130494=DIRECTION('',(0.,1.,0.));
#130495=DIRECTION('center_axis',(0.,1.,0.));
#130496=DIRECTION('ref_axis',(0.,0.,1.));
#130497=DIRECTION('center_axis',(0.,1.,0.));
#130498=DIRECTION('ref_axis',(0.,0.,1.));
#130499=DIRECTION('center_axis',(0.,1.,0.));
#130500=DIRECTION('ref_axis',(0.,0.,1.));
#130501=DIRECTION('',(0.,1.,0.));
#130502=DIRECTION('center_axis',(1.56508116445277E-16,-1.,0.));
#130503=DIRECTION('ref_axis',(1.,1.56508116445277E-16,0.));
#130504=DIRECTION('center_axis',(0.,1.,0.));
#130505=DIRECTION('ref_axis',(0.,0.,1.));
#130506=DIRECTION('center_axis',(-1.56508116445277E-16,1.,0.));
#130507=DIRECTION('ref_axis',(-1.,-1.56508116445277E-16,0.));
#130508=DIRECTION('',(0.,1.,0.));
#130509=DIRECTION('center_axis',(0.,1.,0.));
#130510=DIRECTION('ref_axis',(0.,0.,1.));
#130511=DIRECTION('center_axis',(0.,0.,1.));
#130512=DIRECTION('ref_axis',(1.,0.,0.));
#130513=DIRECTION('center_axis',(0.,0.,1.));
#130514=DIRECTION('ref_axis',(1.,0.,0.));
#130515=DIRECTION('',(0.,0.,1.));
#130516=DIRECTION('center_axis',(0.,0.,1.));
#130517=DIRECTION('ref_axis',(1.,0.,0.));
#130518=DIRECTION('center_axis',(0.,0.,1.));
#130519=DIRECTION('ref_axis',(1.,0.,0.));
#130520=DIRECTION('center_axis',(0.,0.,1.));
#130521=DIRECTION('ref_axis',(1.,0.,0.));
#130522=DIRECTION('',(0.,0.,1.));
#130523=DIRECTION('center_axis',(0.,0.,1.));
#130524=DIRECTION('ref_axis',(1.,0.,0.));
#130525=DIRECTION('center_axis',(0.,0.,1.));
#130526=DIRECTION('ref_axis',(1.,0.,0.));
#130527=DIRECTION('center_axis',(0.,0.,1.));
#130528=DIRECTION('ref_axis',(1.,0.,0.));
#130529=DIRECTION('',(0.,0.,1.));
#130530=DIRECTION('center_axis',(0.,0.,1.));
#130531=DIRECTION('ref_axis',(1.,0.,0.));
#130532=DIRECTION('',(0.,0.,1.));
#130533=DIRECTION('center_axis',(1.,0.,-1.0842021724855E-16));
#130534=DIRECTION('ref_axis',(-1.0842021724855E-16,0.,-1.));
#130535=DIRECTION('',(1.0842021724855E-16,0.,1.));
#130536=DIRECTION('',(0.,1.,0.));
#130537=DIRECTION('',(0.,0.,1.));
#130538=DIRECTION('',(0.,-1.,0.));
#130539=DIRECTION('center_axis',(1.,0.,-1.0842021724855E-16));
#130540=DIRECTION('ref_axis',(-1.0842021724855E-16,0.,-1.));
#130541=DIRECTION('',(0.,0.,1.));
#130542=DIRECTION('',(0.,1.,0.));
#130543=DIRECTION('',(-1.0842021724855E-16,0.,-1.));
#130544=DIRECTION('',(0.,-1.,0.));
#130545=DIRECTION('center_axis',(0.,0.,-1.));
#130546=DIRECTION('ref_axis',(-1.,0.,0.));
#130547=DIRECTION('',(1.,1.56508116445277E-16,0.));
#130548=DIRECTION('',(0.,-1.,0.));
#130549=DIRECTION('',(1.,0.,0.));
#130550=DIRECTION('',(0.,1.,0.));
#130551=DIRECTION('',(-1.,0.,0.));
#130552=DIRECTION('',(0.,-1.,0.));
#130553=DIRECTION('',(-1.,-1.56508116445277E-16,0.));
#130554=DIRECTION('center_axis',(-1.,0.,2.16840434497101E-16));
#130555=DIRECTION('ref_axis',(2.16840434497101E-16,0.,1.));
#130556=DIRECTION('',(2.16840434497101E-16,0.,1.));
#130557=DIRECTION('',(0.,-1.,0.));
#130558=DIRECTION('',(-2.16840434497101E-16,0.,-1.));
#130559=DIRECTION('',(0.,1.,0.));
#130560=DIRECTION('center_axis',(0.,0.,1.));
#130561=DIRECTION('ref_axis',(1.,0.,0.));
#130562=DIRECTION('',(-1.,0.,0.));
#130563=DIRECTION('',(0.,1.,0.));
#130564=DIRECTION('',(1.,1.56508116445277E-16,0.));
#130565=DIRECTION('',(-1.,-1.56508116445277E-16,0.));
#130566=DIRECTION('',(0.,1.,0.));
#130567=DIRECTION('',(1.,0.,0.));
#130568=DIRECTION('',(0.,-1.,0.));
#130569=DIRECTION('center_axis',(0.,1.,0.));
#130570=DIRECTION('ref_axis',(0.,0.,1.));
#130571=DIRECTION('',(1.,0.,0.));
#130572=DIRECTION('',(-2.16840434497101E-16,0.,-1.));
#130573=DIRECTION('',(-1.,0.,0.));
#130574=DIRECTION('',(1.0842021724855E-16,0.,1.));
#130575=DIRECTION('center_axis',(0.,1.,0.));
#130576=DIRECTION('ref_axis',(0.,0.,1.));
#130577=DIRECTION('',(1.,0.,0.));
#130578=DIRECTION('',(2.16840434497101E-16,0.,1.));
#130579=DIRECTION('',(-1.,0.,0.));
#130580=DIRECTION('',(-1.0842021724855E-16,0.,-1.));
#130581=DIRECTION('center_axis',(1.56508116445277E-16,-1.,0.));
#130582=DIRECTION('ref_axis',(1.,1.56508116445277E-16,0.));
#130583=DIRECTION('',(0.707106781186543,1.10667950449189E-16,0.707106781186552));
#130584=DIRECTION('',(-0.707106781186552,-1.1066795044919E-16,0.707106781186543));
#130585=DIRECTION('center_axis',(-1.56508116445277E-16,1.,0.));
#130586=DIRECTION('ref_axis',(-1.,-1.56508116445277E-16,0.));
#130587=DIRECTION('',(-0.707106781186543,-1.10667950449189E-16,-0.707106781186552));
#130588=DIRECTION('',(0.707106781186543,1.10667950449189E-16,-0.707106781186552));
#130589=DIRECTION('center_axis',(0.,0.,1.));
#130590=DIRECTION('ref_axis',(1.,0.,0.));
#130591=DIRECTION('center_axis',(0.,0.,1.));
#130592=DIRECTION('ref_axis',(1.,0.,0.));
#130593=DIRECTION('center_axis',(0.707106781186552,0.,0.707106781186543));
#130594=DIRECTION('ref_axis',(0.,-1.,0.));
#130595=DIRECTION('',(-0.707106781186543,-1.64540693022729E-16,0.707106781186552));
#130596=DIRECTION('center_axis',(0.707106781186543,0.,0.707106781186552));
#130597=DIRECTION('ref_axis',(0.,-1.,0.));
#130598=DIRECTION('',(0.707106781186553,0.,-0.707106781186542));
#130599=DIRECTION('center_axis',(-0.577350269189633,0.57735026918962,-0.577350269189624));
#130600=DIRECTION('ref_axis',(-0.707106781186542,-2.77555756156289E-17,
0.707106781186553));
#130601=DIRECTION('',(5.02745856021284E-15,0.707106781186552,0.707106781186543));
#130602=DIRECTION('',(-0.707106781186546,-0.707106781186549,1.21565128983085E-14));
#130603=DIRECTION('center_axis',(-0.577350269189615,-0.577350269189639,
-0.577350269189623));
#130604=DIRECTION('ref_axis',(-6.38378239159465E-16,0.707106781186538,-0.707106781186557));
#130605=DIRECTION('',(0.707106781186556,-0.707106781186539,1.22847104107341E-14));
#130606=DIRECTION('',(-9.90325783487554E-15,0.707106781186543,-0.707106781186552));
#130607=DIRECTION('center_axis',(0.707106781186552,0.,-0.707106781186543));
#130608=DIRECTION('ref_axis',(0.,-1.,0.));
#130609=DIRECTION('',(0.707106781186543,1.23903709934808E-16,0.707106781186552));
#130610=DIRECTION('center_axis',(-0.707106781186549,0.707106781186546,7.66646708341689E-17));
#130611=DIRECTION('ref_axis',(-1.0842021724855E-16,4.68386162474976E-31,
-1.));
#130612=DIRECTION('',(-0.707106781186546,-0.707106781186549,-1.22206116545212E-14));
#130613=DIRECTION('center_axis',(0.,0.707106781186543,-0.707106781186552));
#130614=DIRECTION('ref_axis',(1.,0.,0.));
#130615=DIRECTION('',(0.,0.707106781186552,0.707106781186543));
#130616=DIRECTION('center_axis',(-0.707106781186552,0.,0.707106781186543));
#130617=DIRECTION('ref_axis',(0.,-1.,0.));
#130618=DIRECTION('',(0.707106781186543,0.,0.707106781186552));
#130619=DIRECTION('',(-0.707106781186543,9.61481343191795E-17,-0.707106781186552));
#130620=DIRECTION('center_axis',(0.,0.707106781186552,0.707106781186543));
#130621=DIRECTION('ref_axis',(-1.,0.,0.));
#130622=DIRECTION('',(9.90325783487536E-15,0.707106781186543,-0.707106781186552));
#130623=DIRECTION('center_axis',(0.707106781186539,0.707106781186556,-7.66646708341678E-17));
#130624=DIRECTION('ref_axis',(1.0842021724855E-16,4.31408307542741E-31,
1.));
#130625=DIRECTION('',(0.707106781186556,-0.707106781186539,-2.3796250225573E-15));
#130626=DIRECTION('center_axis',(0.707106781186552,0.,-0.707106781186543));
#130627=DIRECTION('ref_axis',(0.,-1.,0.));
#130628=DIRECTION('',(-0.707106781186542,4.06369830879181E-17,-0.707106781186553));
#130629=DIRECTION('center_axis',(-0.577350269189633,0.57735026918962,0.577350269189625));
#130630=DIRECTION('ref_axis',(0.707106781186543,-1.38777878078144E-16,0.707106781186553));
#130631=DIRECTION('',(-4.90355485027803E-15,-0.707106781186552,0.707106781186543));
#130632=DIRECTION('center_axis',(0.577350269189634,0.577350269189618,-0.577350269189626));
#130633=DIRECTION('ref_axis',(-0.707106781186543,-1.38777878078144E-16,
-0.707106781186553));
#130634=DIRECTION('',(-0.707106781186543,0.707106781186552,-9.90508538817675E-15));
#130635=DIRECTION('center_axis',(0.577350269189626,-0.577350269189634,-0.577350269189618));
#130636=DIRECTION('ref_axis',(0.707106781186553,0.707106781186543,1.38777878078144E-16));
#130637=DIRECTION('',(0.707106781186552,0.707106781186543,-1.19609907444045E-16));
#130638=DIRECTION('center_axis',(-0.577350269189623,-0.577350269189639,
0.577350269189615));
#130639=DIRECTION('ref_axis',(0.707106781186557,-0.707106781186538,-6.38378239159465E-16));
#130640=DIRECTION('',(1.96142194011124E-14,-0.707106781186543,-0.707106781186552));
#130641=DIRECTION('center_axis',(0.,0.707106781186543,0.707106781186552));
#130642=DIRECTION('ref_axis',(-1.,0.,0.));
#130643=DIRECTION('',(-1.46829089752187E-14,-0.707106781186552,0.707106781186543));
#130644=DIRECTION('center_axis',(0.707106781186552,0.707106781186543,-1.53329341668338E-16));
#130645=DIRECTION('ref_axis',(2.16840434497101E-16,-6.28623533847994E-31,
1.));
#130646=DIRECTION('',(-0.707106781186542,0.707106781186553,2.77555756156289E-17));
#130647=DIRECTION('center_axis',(-0.707106781186543,0.707106781186552,1.53329341668336E-16));
#130648=DIRECTION('ref_axis',(-2.16840434497101E-16,-6.77927340424307E-31,
-1.));
#130649=DIRECTION('',(0.707106781186552,0.707106781186543,9.90508538817668E-15));
#130650=DIRECTION('center_axis',(0.,0.707106781186552,-0.707106781186543));
#130651=DIRECTION('ref_axis',(1.,0.,0.));
#130652=DIRECTION('',(4.77965114034336E-15,-0.707106781186543,-0.707106781186552));
#130653=DIRECTION('center_axis',(0.577350269189624,0.577350269189617,0.577350269189636));
#130654=DIRECTION('ref_axis',(0.707106781186555,-2.22044604925031E-16,-0.70710678118654));
#130655=DIRECTION('',(-0.707106781186555,6.83925587035508E-17,0.70710678118654));
#130656=DIRECTION('center_axis',(0.577350269189617,-0.577350269189632,0.577350269189628));
#130657=DIRECTION('ref_axis',(1.11022302462516E-16,-0.707106781186545,-0.70710678118655));
#130658=DIRECTION('',(0.707106781186555,5.55111512312578E-17,-0.70710678118654));
#130659=DIRECTION('center_axis',(-0.70710678118654,0.,-0.707106781186555));
#130660=DIRECTION('ref_axis',(0.,-1.,0.));
#458995=CARTESIAN_POINT('',(0.,0.,0.));
#458996=CARTESIAN_POINT('Origin',(5.50000000000001,0.,-6.93889390390723E-15));
#458997=CARTESIAN_POINT('',(5.50000000000001,0.,-3.00000000000001));
#458998=CARTESIAN_POINT('Origin',(5.50000000000001,0.,-6.93889390390723E-15));
#458999=CARTESIAN_POINT('',(5.50000000000001,11.5,-3.00000000000001));
#459000=CARTESIAN_POINT('',(5.50000000000001,0.,-3.00000000000001));
#459001=CARTESIAN_POINT('Origin',(5.50000000000001,11.5,-6.93889390390723E-15));
#459002=CARTESIAN_POINT('Origin',(-7.5,0.,-6.93889390390723E-15));
#459003=CARTESIAN_POINT('',(-7.5,0.,-1.50000000000001));
#459004=CARTESIAN_POINT('Origin',(-7.5,0.,-6.93889390390723E-15));
#459005=CARTESIAN_POINT('',(-7.5,3.5,-1.50000000000001));
#459006=CARTESIAN_POINT('',(-7.5,0.,-1.50000000000001));
#459007=CARTESIAN_POINT('Origin',(-7.5,3.5,-6.93889390390723E-15));
#459008=CARTESIAN_POINT('Origin',(-7.5,0.,-6.93889390390723E-15));
#459009=CARTESIAN_POINT('',(-7.5,4.5,-1.50000000000001));
#459010=CARTESIAN_POINT('Origin',(-7.5,4.5,-6.93889390390723E-15));
#459011=CARTESIAN_POINT('',(-7.5,11.5,-1.50000000000001));
#459012=CARTESIAN_POINT('',(-7.5,0.,-1.50000000000001));
#459013=CARTESIAN_POINT('Origin',(-7.5,11.5,-6.93889390390723E-15));
#459014=CARTESIAN_POINT('Origin',(8.00000000000001,2.,3.49999999999999));
#459015=CARTESIAN_POINT('',(7.25000000000001,2.,3.49999999999999));
#459016=CARTESIAN_POINT('Origin',(8.00000000000001,2.,3.49999999999999));
#459017=CARTESIAN_POINT('',(7.25000000000001,2.,7.99999999999999));
#459018=CARTESIAN_POINT('',(7.25000000000001,2.,3.49999999999999));
#459019=CARTESIAN_POINT('Origin',(8.00000000000001,2.,7.99999999999999));
#459020=CARTESIAN_POINT('Origin',(6.50000000000001,4.8,4.49999999999999));
#459021=CARTESIAN_POINT('',(5.00000000000001,4.8,4.49999999999999));
#459022=CARTESIAN_POINT('Origin',(6.50000000000001,4.8,4.49999999999999));
#459023=CARTESIAN_POINT('',(5.00000000000001,4.8,7.99999999999999));
#459024=CARTESIAN_POINT('',(5.00000000000001,4.8,4.49999999999999));
#459025=CARTESIAN_POINT('Origin',(6.50000000000001,4.8,7.99999999999999));
#459026=CARTESIAN_POINT('Origin',(-1.49999999999999,4.,-8.00000000000001));
#459027=CARTESIAN_POINT('',(-4.4580398915498,3.5,-8.00000000000001));
#459028=CARTESIAN_POINT('',(-4.4580398915498,4.5,-8.00000000000001));
#459029=CARTESIAN_POINT('Origin',(-1.49999999999999,4.,-8.00000000000001));
#459030=CARTESIAN_POINT('',(-4.4580398915498,3.5,7.99999999999999));
#459031=CARTESIAN_POINT('',(-4.4580398915498,3.5,-8.00000000000001));
#459032=CARTESIAN_POINT('',(-4.4580398915498,4.5,7.99999999999999));
#459033=CARTESIAN_POINT('Origin',(-1.49999999999999,4.,7.99999999999999));
#459034=CARTESIAN_POINT('',(-4.4580398915498,4.5,-8.00000000000001));
#459035=CARTESIAN_POINT('Origin',(-10.,11.5,-8.00000000000001));
#459036=CARTESIAN_POINT('',(-10.,0.249999999999997,-7.75000000000001));
#459037=CARTESIAN_POINT('',(-10.,0.249999999999997,7.74999999999999));
#459038=CARTESIAN_POINT('',(-10.,0.249999999999997,-8.00000000000001));
#459039=CARTESIAN_POINT('',(-10.,3.5,7.74999999999999));
#459040=CARTESIAN_POINT('',(-10.,11.5,7.74999999999999));
#459041=CARTESIAN_POINT('',(-10.,3.5,-7.75000000000001));
#459042=CARTESIAN_POINT('',(-10.,3.5,-8.00000000000001));
#459043=CARTESIAN_POINT('',(-10.,11.5,-7.75000000000001));
#459044=CARTESIAN_POINT('Origin',(-10.,11.5,-8.00000000000001));
#459045=CARTESIAN_POINT('',(-10.,4.5,-7.75000000000001));
#459046=CARTESIAN_POINT('',(-10.,4.5,7.74999999999999));
#459047=CARTESIAN_POINT('',(-10.,4.5,-8.00000000000001));
#459048=CARTESIAN_POINT('',(-10.,11.25,7.74999999999999));
#459049=CARTESIAN_POINT('',(-10.,11.5,7.74999999999999));
#459050=CARTESIAN_POINT('',(-10.,11.25,-7.75000000000001));
#459051=CARTESIAN_POINT('',(-10.,11.25,-8.00000000000001));
#459052=CARTESIAN_POINT('',(-10.,11.5,-7.75000000000001));
#459053=CARTESIAN_POINT('Origin',(-10.,11.5,7.99999999999999));
#459054=CARTESIAN_POINT('',(-9.75,3.5,7.99999999999999));
#459055=CARTESIAN_POINT('',(-10.,3.5,7.99999999999999));
#459056=CARTESIAN_POINT('',(-9.75,0.249999999999997,7.99999999999999));
#459057=CARTESIAN_POINT('',(-9.75,11.5,7.99999999999999));
#459058=CARTESIAN_POINT('',(9.75000000000001,0.249999999999997,7.99999999999999));
#459059=CARTESIAN_POINT('',(-10.,0.249999999999997,7.99999999999999));
#459060=CARTESIAN_POINT('',(9.75000000000001,11.25,7.99999999999999));
#459061=CARTESIAN_POINT('',(9.75000000000001,11.5,7.99999999999999));
#459062=CARTESIAN_POINT('',(-9.75,11.25,7.99999999999999));
#459063=CARTESIAN_POINT('',(-10.,11.25,7.99999999999999));
#459064=CARTESIAN_POINT('',(-9.75,4.5,7.99999999999999));
#459065=CARTESIAN_POINT('',(-9.75,11.5,7.99999999999999));
#459066=CARTESIAN_POINT('',(-4.4580398915498,4.5,7.99999999999999));
#459067=CARTESIAN_POINT('Origin',(10.,11.5,-8.00000000000001));
#459068=CARTESIAN_POINT('',(10.,11.25,-7.75000000000001));
#459069=CARTESIAN_POINT('',(10.,11.25,7.75));
#459070=CARTESIAN_POINT('',(10.,11.25,7.99999999999999));
#459071=CARTESIAN_POINT('',(10.,0.249999999999997,7.75));
#459072=CARTESIAN_POINT('',(10.,11.5,7.75));
#459073=CARTESIAN_POINT('',(10.,0.249999999999997,-7.75000000000001));
#459074=CARTESIAN_POINT('',(10.,0.249999999999997,-8.00000000000001));
#459075=CARTESIAN_POINT('',(10.,11.5,-7.75000000000001));
#459076=CARTESIAN_POINT('Origin',(-10.,11.5,-8.00000000000001));
#459077=CARTESIAN_POINT('',(9.75000000000001,0.249999999999997,-8.00000000000001));
#459078=CARTESIAN_POINT('',(-9.75,0.249999999999997,-8.00000000000001));
#459079=CARTESIAN_POINT('',(-10.,0.249999999999997,-8.00000000000001));
#459080=CARTESIAN_POINT('',(-9.75,3.5,-8.00000000000001));
#459081=CARTESIAN_POINT('',(-9.75,11.5,-8.00000000000001));
#459082=CARTESIAN_POINT('',(-10.,3.5,-8.00000000000001));
#459083=CARTESIAN_POINT('',(-9.75,4.5,-8.00000000000001));
#459084=CARTESIAN_POINT('',(-4.4580398915498,4.5,-8.00000000000001));
#459085=CARTESIAN_POINT('',(-9.75,11.25,-8.00000000000001));
#459086=CARTESIAN_POINT('',(-9.75,11.5,-8.00000000000001));
#459087=CARTESIAN_POINT('',(9.75000000000001,11.25,-8.00000000000001));
#459088=CARTESIAN_POINT('',(10.,11.25,-8.00000000000001));
#459089=CARTESIAN_POINT('',(9.75000000000001,11.5,-8.00000000000001));
#459090=CARTESIAN_POINT('Origin',(0.,11.5,0.));
#459091=CARTESIAN_POINT('',(-9.75,11.5,7.75));
#459092=CARTESIAN_POINT('',(9.75000000000001,11.5,7.75));
#459093=CARTESIAN_POINT('',(10.,11.5,7.75));
#459094=CARTESIAN_POINT('',(9.75000000000001,11.5,-7.75000000000001));
#459095=CARTESIAN_POINT('',(9.75000000000001,11.5,-8.00000000000001));
#459096=CARTESIAN_POINT('',(-9.75,11.5,-7.75000000000001));
#459097=CARTESIAN_POINT('',(-10.,11.5,-7.75000000000001));
#459098=CARTESIAN_POINT('',(-9.75,11.5,7.99999999999999));
#459099=CARTESIAN_POINT('Origin',(0.,0.,0.));
#459100=CARTESIAN_POINT('',(-9.74999999999999,0.,-7.75000000000001));
#459101=CARTESIAN_POINT('',(9.75,0.,-7.75000000000001));
#459102=CARTESIAN_POINT('',(0.,0.,-7.75000000000001));
#459103=CARTESIAN_POINT('',(9.75000000000001,0.,7.74999999999999));
#459104=CARTESIAN_POINT('',(9.75000000000001,0.,-2.11419423634673E-15));
#459105=CARTESIAN_POINT('',(-9.74999999999999,0.,7.74999999999999));
#459106=CARTESIAN_POINT('',(0.,0.,7.74999999999999));
#459107=CARTESIAN_POINT('',(-9.74999999999999,0.,1.05709711817337E-15));
#459108=CARTESIAN_POINT('Origin',(-10.,3.5,-8.00000000000001));
#459109=CARTESIAN_POINT('',(-9.75,3.5,7.99999999999999));
#459110=CARTESIAN_POINT('',(-10.,3.5,-7.75000000000001));
#459111=CARTESIAN_POINT('Origin',(-4.4580398915498,4.5,-8.00000000000001));
#459112=CARTESIAN_POINT('',(-9.75,4.5,7.99999999999999));
#459113=CARTESIAN_POINT('',(-10.,4.5,-7.75000000000001));
#459114=CARTESIAN_POINT('Origin',(6.50000000000001,4.8,4.49999999999999));
#459115=CARTESIAN_POINT('Origin',(8.00000000000001,2.,3.49999999999999));
#459116=CARTESIAN_POINT('Origin',(-10.,11.5,-7.75000000000001));
#459117=CARTESIAN_POINT('',(-9.75,11.25,-8.00000000000001));
#459118=CARTESIAN_POINT('Origin',(-10.,11.5,-7.75000000000001));
#459119=CARTESIAN_POINT('',(-10.,0.249999999999997,-7.75000000000001));
#459120=CARTESIAN_POINT('Origin',(-9.75,11.25,-8.00000000000001));
#459121=CARTESIAN_POINT('',(-9.75,11.25,-8.00000000000001));
#459122=CARTESIAN_POINT('',(-9.875,11.375,-7.75000000000001));
#459123=CARTESIAN_POINT('Origin',(-10.,0.249999999999997,-7.75000000000001));
#459124=CARTESIAN_POINT('',(-10.,0.249999999999997,-7.75000000000001));
#459125=CARTESIAN_POINT('',(-9.74999999999999,0.125,-7.87500000000001));
#459126=CARTESIAN_POINT('Origin',(-9.75,11.5,7.99999999999999));
#459127=CARTESIAN_POINT('',(-10.,11.25,7.74999999999999));
#459128=CARTESIAN_POINT('Origin',(-9.75,11.5,1.05709711817337E-15));
#459129=CARTESIAN_POINT('',(-10.,11.25,7.74999999999999));
#459130=CARTESIAN_POINT('Origin',(0.,11.5,-7.75000000000001));
#459131=CARTESIAN_POINT('',(9.75000000000001,11.5,-7.75000000000001));
#459132=CARTESIAN_POINT('Origin',(9.75000000000001,11.5,-8.00000000000001));
#459133=CARTESIAN_POINT('',(10.,0.249999999999997,-7.75000000000001));
#459134=CARTESIAN_POINT('',(9.87500000000001,11.25,-7.87500000000001));
#459135=CARTESIAN_POINT('Origin',(-10.,0.249999999999997,-8.00000000000001));
#459136=CARTESIAN_POINT('',(9.75000000000001,0.124999999999998,-7.87500000000001));
#459137=CARTESIAN_POINT('Origin',(-10.,0.249999999999997,-8.00000000000001));
#459138=CARTESIAN_POINT('',(-9.87499999999999,0.124999999999999,7.74999999999999));
#459139=CARTESIAN_POINT('Origin',(-9.75,11.5,7.99999999999999));
#459140=CARTESIAN_POINT('',(-9.75,0.249999999999997,7.99999999999999));
#459141=CARTESIAN_POINT('Origin',(-10.,11.25,7.74999999999999));
#459142=CARTESIAN_POINT('',(-9.75,11.375,7.875));
#459143=CARTESIAN_POINT('Origin',(9.75000000000001,11.5,-7.75000000000001));
#459144=CARTESIAN_POINT('',(9.75000000000001,11.5,-7.75000000000001));
#459145=CARTESIAN_POINT('Origin',(10.,0.249999999999997,-7.75000000000001));
#459146=CARTESIAN_POINT('',(10.,0.249999999999997,-7.75000000000001));
#459147=CARTESIAN_POINT('Origin',(-9.75,0.249999999999997,7.99999999999999));
#459148=CARTESIAN_POINT('',(-9.75,0.249999999999997,7.99999999999999));
#459149=CARTESIAN_POINT('Origin',(0.,11.5,7.75));
#459150=CARTESIAN_POINT('',(9.75000000000001,11.25,7.99999999999999));
#459151=CARTESIAN_POINT('Origin',(9.75000000000001,11.5,-2.11419423634674E-15));
#459152=CARTESIAN_POINT('',(9.87500000000001,11.375,7.75));
#459153=CARTESIAN_POINT('Origin',(10.,0.249999999999997,-8.00000000000001));
#459154=CARTESIAN_POINT('',(10.,0.249999999999997,7.75));
#459155=CARTESIAN_POINT('Origin',(-10.,0.249999999999997,7.99999999999999));
#459156=CARTESIAN_POINT('',(9.75000000000001,0.124999999999998,7.87499999999999));
#459157=CARTESIAN_POINT('Origin',(9.75000000000001,11.25,7.99999999999999));
#459158=CARTESIAN_POINT('',(9.75000000000001,11.25,7.99999999999999));
#459159=CARTESIAN_POINT('Origin',(10.,0.249999999999997,7.75));
#459160=CARTESIAN_POINT('',(10.,0.249999999999997,7.75));
#459161=CARTESIAN_POINT('Origin',(10.,11.5,7.75));
#459215=UNCERTAINTY_MEASURE_WITH_UNIT(LENGTH_MEASURE(0.01),#459243,
'DISTANCE_ACCURACY_VALUE',
'Maximum model space distance between geometric entities at asserted c
onnectivities');
#459216=UNCERTAINTY_MEASURE_WITH_UNIT(LENGTH_MEASURE(0.01),#459243,
'DISTANCE_ACCURACY_VALUE',
'Maximum model space distance between geometric entities at asserted c
onnectivities');
#459241=(
GEOMETRIC_REPRESENTATION_CONTEXT(3)
GLOBAL_UNCERTAINTY_ASSIGNED_CONTEXT((#459215))
GLOBAL_UNIT_ASSIGNED_CONTEXT((#459243,#459245,#459246))
REPRESENTATION_CONTEXT('','3D')
);
#459242=(
GEOMETRIC_REPRESENTATION_CONTEXT(3)
GLOBAL_UNCERTAINTY_ASSIGNED_CONTEXT((#459216))
GLOBAL_UNIT_ASSIGNED_CONTEXT((#459243,#459245,#459246))
REPRESENTATION_CONTEXT('','3D')
);
#459243=(
LENGTH_UNIT()
NAMED_UNIT(*)
SI_UNIT(.MILLI.,.METRE.)
);
#459245=(
NAMED_UNIT(*)
PLANE_ANGLE_UNIT()
SI_UNIT($,.RADIAN.)
);
#459246=(
NAMED_UNIT(*)
SI_UNIT($,.STERADIAN.)
SOLID_ANGLE_UNIT()
);
#459271=SHAPE_DEFINITION_REPRESENTATION(#459298,#459352);
#459298=PRODUCT_DEFINITION_SHAPE('',$,#459378);
#459352=SHAPE_REPRESENTATION('',(#105494),#459241);
#459353=PRODUCT_DEFINITION_CONTEXT('part definition',#459430,'design');
#459378=PRODUCT_DEFINITION('Hotend Heater Block','Hotend Heater Block',
#459403,#459353);
#459403=PRODUCT_DEFINITION_FORMATION('',$,#459456);
#459430=APPLICATION_CONTEXT(
'Core Data for Automotive Mechanical Design Process');
#459431=PRODUCT_CONTEXT('part definition',#459430,'mechanical');
#459456=PRODUCT('Hotend Heater Block','Hotend Heater Block',$,(#459431));
#459499=COLOUR_RGB('Dark Blue',0.08,0.2,0.34);
#459500=FILL_AREA_STYLE_COLOUR('',#459499);
#459501=FILL_AREA_STYLE('',(#459500));
#459502=SURFACE_STYLE_FILL_AREA(#459501);
#459503=SURFACE_SIDE_STYLE('',(#459502));
#459504=SURFACE_STYLE_USAGE(.BOTH.,#459503);
#459505=PRESENTATION_STYLE_ASSIGNMENT((#459504));
ENDSEC;
END-ISO-10303-21;
